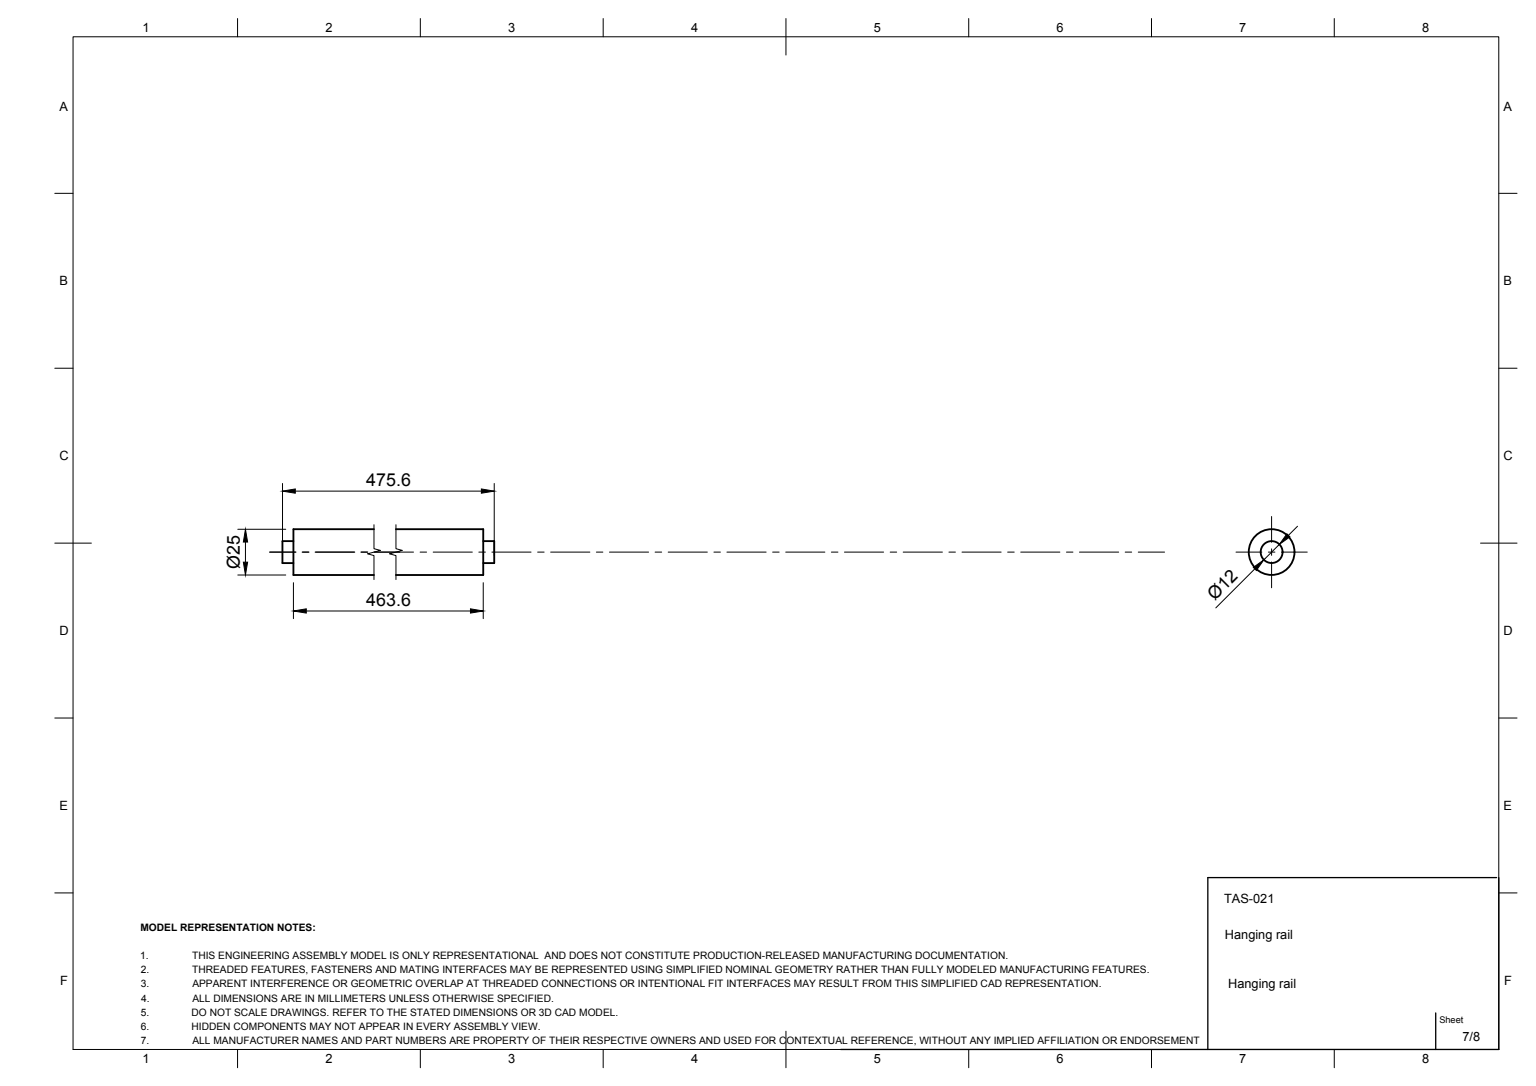
ISO-10303-21;
HEADER;
/* Generated by software containing ST-Developer
 * from STEP Tools, Inc. (www.steptools.com) 
 */

FILE_DESCRIPTION(
/* description */ (''),
/* implementation_level */ '2;1');

FILE_NAME(
/* name */ 'Hanging rail.step',
/* time_stamp */ '2026-11-15T17:48:08-08:00',
/* author */ (''),
/* organization */ (''),
/* preprocessor_version */ 'ST-DEVELOPER v20.2',
/* originating_system */ 'Autodesk Translation Framework v15.17.0.0',
/* authorisation */ '');

FILE_SCHEMA (('AUTOMOTIVE_DESIGN { 1 0 10303 214 3 1 1 }'));
ENDSEC;

DATA;
#10=MECHANICAL_DESIGN_GEOMETRIC_PRESENTATION_REPRESENTATION('',(#143),#2097);
#131=SHAPE_REPRESENTATION_RELATIONSHIP('SRR','None',#2150,#137);
#137=ADVANCED_BREP_SHAPE_REPRESENTATION('',(#149),#2095);
#143=STYLED_ITEM('',(#2189),#149);
#149=MANIFOLD_SOLID_BREP('Body1',#1197);
#157=FACE_BOUND('',#349,.T.);
#158=FACE_BOUND('',#351,.T.);
#209=PLANE('',#1343);
#210=PLANE('',#1347);
#211=PLANE('',#1351);
#212=PLANE('',#1352);
#271=FACE_OUTER_BOUND('',#343,.T.);
#272=FACE_OUTER_BOUND('',#344,.T.);
#273=FACE_OUTER_BOUND('',#345,.T.);
#274=FACE_OUTER_BOUND('',#346,.T.);
#275=FACE_OUTER_BOUND('',#347,.T.);
#276=FACE_OUTER_BOUND('',#348,.T.);
#277=FACE_OUTER_BOUND('',#350,.T.);
#343=EDGE_LOOP('',(#1093,#1094,#1095,#1096));
#344=EDGE_LOOP('',(#1097));
#345=EDGE_LOOP('',(#1098,#1099,#1100,#1101));
#346=EDGE_LOOP('',(#1102));
#347=EDGE_LOOP('',(#1103,#1104,#1105,#1106));
#348=EDGE_LOOP('',(#1107));
#349=EDGE_LOOP('',(#1108));
#350=EDGE_LOOP('',(#1109));
#351=EDGE_LOOP('',(#1110));
#469=LINE('',#2026,#587);
#470=LINE('',#2033,#588);
#471=LINE('',#2040,#589);
#587=VECTOR('',#1654,0.6);
#588=VECTOR('',#1663,0.6);
#589=VECTOR('',#1672,1.25);
#603=CIRCLE('',#1341,0.6);
#604=CIRCLE('',#1342,0.6);
#605=CIRCLE('',#1345,0.6);
#606=CIRCLE('',#1346,0.6);
#607=CIRCLE('',#1349,1.25);
#608=CIRCLE('',#1350,1.25);
#695=VERTEX_POINT('',#2023);
#696=VERTEX_POINT('',#2025);
#697=VERTEX_POINT('',#2030);
#698=VERTEX_POINT('',#2032);
#699=VERTEX_POINT('',#2037);
#700=VERTEX_POINT('',#2039);
#829=EDGE_CURVE('',#695,#695,#603,.T.);
#830=EDGE_CURVE('',#695,#696,#469,.T.);
#831=EDGE_CURVE('',#696,#696,#604,.T.);
#832=EDGE_CURVE('',#697,#697,#605,.T.);
#833=EDGE_CURVE('',#697,#698,#470,.T.);
#834=EDGE_CURVE('',#698,#698,#606,.T.);
#835=EDGE_CURVE('',#699,#699,#607,.T.);
#836=EDGE_CURVE('',#699,#700,#471,.T.);
#837=EDGE_CURVE('',#700,#700,#608,.T.);
#1093=ORIENTED_EDGE('',*,*,#829,.F.);
#1094=ORIENTED_EDGE('',*,*,#830,.T.);
#1095=ORIENTED_EDGE('',*,*,#831,.F.);
#1096=ORIENTED_EDGE('',*,*,#830,.F.);
#1097=ORIENTED_EDGE('',*,*,#829,.T.);
#1098=ORIENTED_EDGE('',*,*,#832,.F.);
#1099=ORIENTED_EDGE('',*,*,#833,.T.);
#1100=ORIENTED_EDGE('',*,*,#834,.T.);
#1101=ORIENTED_EDGE('',*,*,#833,.F.);
#1102=ORIENTED_EDGE('',*,*,#834,.F.);
#1103=ORIENTED_EDGE('',*,*,#835,.F.);
#1104=ORIENTED_EDGE('',*,*,#836,.T.);
#1105=ORIENTED_EDGE('',*,*,#837,.T.);
#1106=ORIENTED_EDGE('',*,*,#836,.F.);
#1107=ORIENTED_EDGE('',*,*,#835,.T.);
#1108=ORIENTED_EDGE('',*,*,#831,.T.);
#1109=ORIENTED_EDGE('',*,*,#837,.F.);
#1110=ORIENTED_EDGE('',*,*,#832,.T.);
#1123=CYLINDRICAL_SURFACE('',#1340,0.6);
#1124=CYLINDRICAL_SURFACE('',#1344,0.6);
#1125=CYLINDRICAL_SURFACE('',#1348,1.25);
#1183=ADVANCED_FACE('',(#271),#1123,.T.);
#1184=ADVANCED_FACE('',(#272),#209,.T.);
#1185=ADVANCED_FACE('',(#273),#1124,.T.);
#1186=ADVANCED_FACE('',(#274),#210,.F.);
#1187=ADVANCED_FACE('',(#275),#1125,.T.);
#1188=ADVANCED_FACE('',(#276,#157),#211,.T.);
#1189=ADVANCED_FACE('',(#277,#158),#212,.F.);
#1197=CLOSED_SHELL('',(#1183,#1184,#1185,#1186,#1187,#1188,#1189));
#1339=AXIS2_PLACEMENT_3D('',#2021,#1648,#1649);
#1340=AXIS2_PLACEMENT_3D('',#2022,#1650,#1651);
#1341=AXIS2_PLACEMENT_3D('',#2024,#1652,#1653);
#1342=AXIS2_PLACEMENT_3D('',#2027,#1655,#1656);
#1343=AXIS2_PLACEMENT_3D('',#2028,#1657,#1658);
#1344=AXIS2_PLACEMENT_3D('',#2029,#1659,#1660);
#1345=AXIS2_PLACEMENT_3D('',#2031,#1661,#1662);
#1346=AXIS2_PLACEMENT_3D('',#2034,#1664,#1665);
#1347=AXIS2_PLACEMENT_3D('',#2035,#1666,#1667);
#1348=AXIS2_PLACEMENT_3D('',#2036,#1668,#1669);
#1349=AXIS2_PLACEMENT_3D('',#2038,#1670,#1671);
#1350=AXIS2_PLACEMENT_3D('',#2041,#1673,#1674);
#1351=AXIS2_PLACEMENT_3D('',#2042,#1675,#1676);
#1352=AXIS2_PLACEMENT_3D('',#2043,#1677,#1678);
#1648=DIRECTION('axis',(0.,0.,1.));
#1649=DIRECTION('refdir',(1.,0.,0.));
#1650=DIRECTION('center_axis',(0.,0.,1.));
#1651=DIRECTION('ref_axis',(1.,0.,0.));
#1652=DIRECTION('center_axis',(0.,0.,1.));
#1653=DIRECTION('ref_axis',(1.,0.,0.));
#1654=DIRECTION('',(0.,0.,-1.));
#1655=DIRECTION('center_axis',(0.,0.,-1.));
#1656=DIRECTION('ref_axis',(1.,0.,0.));
#1657=DIRECTION('center_axis',(0.,0.,1.));
#1658=DIRECTION('ref_axis',(1.,0.,0.));
#1659=DIRECTION('center_axis',(0.,0.,1.));
#1660=DIRECTION('ref_axis',(1.,0.,0.));
#1661=DIRECTION('center_axis',(0.,0.,1.));
#1662=DIRECTION('ref_axis',(1.,0.,0.));
#1663=DIRECTION('',(0.,0.,-1.));
#1664=DIRECTION('center_axis',(0.,0.,1.));
#1665=DIRECTION('ref_axis',(1.,0.,0.));
#1666=DIRECTION('center_axis',(0.,0.,1.));
#1667=DIRECTION('ref_axis',(1.,0.,0.));
#1668=DIRECTION('center_axis',(0.,0.,1.));
#1669=DIRECTION('ref_axis',(1.,0.,0.));
#1670=DIRECTION('center_axis',(0.,0.,1.));
#1671=DIRECTION('ref_axis',(1.,0.,0.));
#1672=DIRECTION('',(0.,0.,-1.));
#1673=DIRECTION('center_axis',(0.,0.,1.));
#1674=DIRECTION('ref_axis',(1.,0.,0.));
#1675=DIRECTION('center_axis',(0.,0.,1.));
#1676=DIRECTION('ref_axis',(1.,0.,0.));
#1677=DIRECTION('center_axis',(0.,0.,1.));
#1678=DIRECTION('ref_axis',(1.,0.,0.));
#2021=CARTESIAN_POINT('',(0.,0.,0.));
#2022=CARTESIAN_POINT('Origin',(0.,0.,46.36));
#2023=CARTESIAN_POINT('',(-0.6,-7.34788079488412E-17,46.96));
#2024=CARTESIAN_POINT('Origin',(0.,0.,46.96));
#2025=CARTESIAN_POINT('',(-0.6,-7.34788079488412E-17,46.36));
#2026=CARTESIAN_POINT('',(-0.6,-7.34788079488412E-17,46.36));
#2027=CARTESIAN_POINT('Origin',(0.,0.,46.36));
#2028=CARTESIAN_POINT('Origin',(0.,0.,46.96));
#2029=CARTESIAN_POINT('Origin',(0.,0.,-0.6));
#2030=CARTESIAN_POINT('',(-0.6,-7.34788079488412E-17,0.));
#2031=CARTESIAN_POINT('Origin',(0.,0.,0.));
#2032=CARTESIAN_POINT('',(-0.6,-7.34788079488412E-17,-0.6));
#2033=CARTESIAN_POINT('',(-0.6,-7.34788079488412E-17,-0.6));
#2034=CARTESIAN_POINT('Origin',(0.,0.,-0.6));
#2035=CARTESIAN_POINT('Origin',(0.,0.,-0.6));
#2036=CARTESIAN_POINT('Origin',(0.,0.,0.));
#2037=CARTESIAN_POINT('',(-1.25,-1.53080849893419E-16,46.36));
#2038=CARTESIAN_POINT('Origin',(0.,0.,46.36));
#2039=CARTESIAN_POINT('',(-1.25,-1.53080849893419E-16,0.));
#2040=CARTESIAN_POINT('',(-1.25,-1.53080849893419E-16,0.));
#2041=CARTESIAN_POINT('Origin',(0.,0.,0.));
#2042=CARTESIAN_POINT('Origin',(0.,0.,46.36));
#2043=CARTESIAN_POINT('Origin',(0.,0.,0.));
#2087=UNCERTAINTY_MEASURE_WITH_UNIT(LENGTH_MEASURE(0.001),#2098,
'DISTANCE_ACCURACY_VALUE',
'Maximum model space distance between geometric entities at asserted c
onnectivities');
#2089=UNCERTAINTY_MEASURE_WITH_UNIT(LENGTH_MEASURE(0.001),#2098,
'DISTANCE_ACCURACY_VALUE',
'Maximum model space distance between geometric entities at asserted c
onnectivities');
#2095=(
GEOMETRIC_REPRESENTATION_CONTEXT(3)
GLOBAL_UNCERTAINTY_ASSIGNED_CONTEXT((#2087))
GLOBAL_UNIT_ASSIGNED_CONTEXT((#2098,#2100,#2101))
REPRESENTATION_CONTEXT('','3D')
);
#2097=(
GEOMETRIC_REPRESENTATION_CONTEXT(3)
GLOBAL_UNCERTAINTY_ASSIGNED_CONTEXT((#2089))
GLOBAL_UNIT_ASSIGNED_CONTEXT((#2098,#2100,#2101))
REPRESENTATION_CONTEXT('','3D')
);
#2098=(
LENGTH_UNIT()
NAMED_UNIT(*)
SI_UNIT(.CENTI.,.METRE.)
);
#2100=(
NAMED_UNIT(*)
PLANE_ANGLE_UNIT()
SI_UNIT($,.RADIAN.)
);
#2101=(
NAMED_UNIT(*)
SI_UNIT($,.STERADIAN.)
SOLID_ANGLE_UNIT()
);
#2107=SHAPE_DEFINITION_REPRESENTATION(#2114,#2150);
#2114=PRODUCT_DEFINITION_SHAPE('',$,#2158);
#2150=SHAPE_REPRESENTATION('',(#1339),#2095);
#2152=PRODUCT_DEFINITION_CONTEXT('part definition',#2175,'design');
#2158=PRODUCT_DEFINITION('Hanging rail','Hanging rail',#2165,#2152);
#2165=PRODUCT_DEFINITION_FORMATION('',$,#2182);
#2175=APPLICATION_CONTEXT(
'Core Data for Automotive Mechanical Design Process');
#2176=PRODUCT_CONTEXT('part definition',#2175,'mechanical');
#2182=PRODUCT('Hanging rail','Hanging rail',$,(#2176));
#2189=PRESENTATION_STYLE_ASSIGNMENT((#2196));
#2196=SURFACE_STYLE_USAGE(.BOTH.,#2203);
#2203=SURFACE_SIDE_STYLE('',(#2210));
#2210=SURFACE_STYLE_FILL_AREA(#2217);
#2217=FILL_AREA_STYLE('Hanging rail finish',(#2224));
#2224=FILL_AREA_STYLE_COLOUR('Hanging rail finish',#2231);
#2231=COLOUR_RGB('Hanging rail finish',0.607843137254902,0.647058823529412,
0.701960784313725);
ENDSEC;
END-ISO-10303-21;
